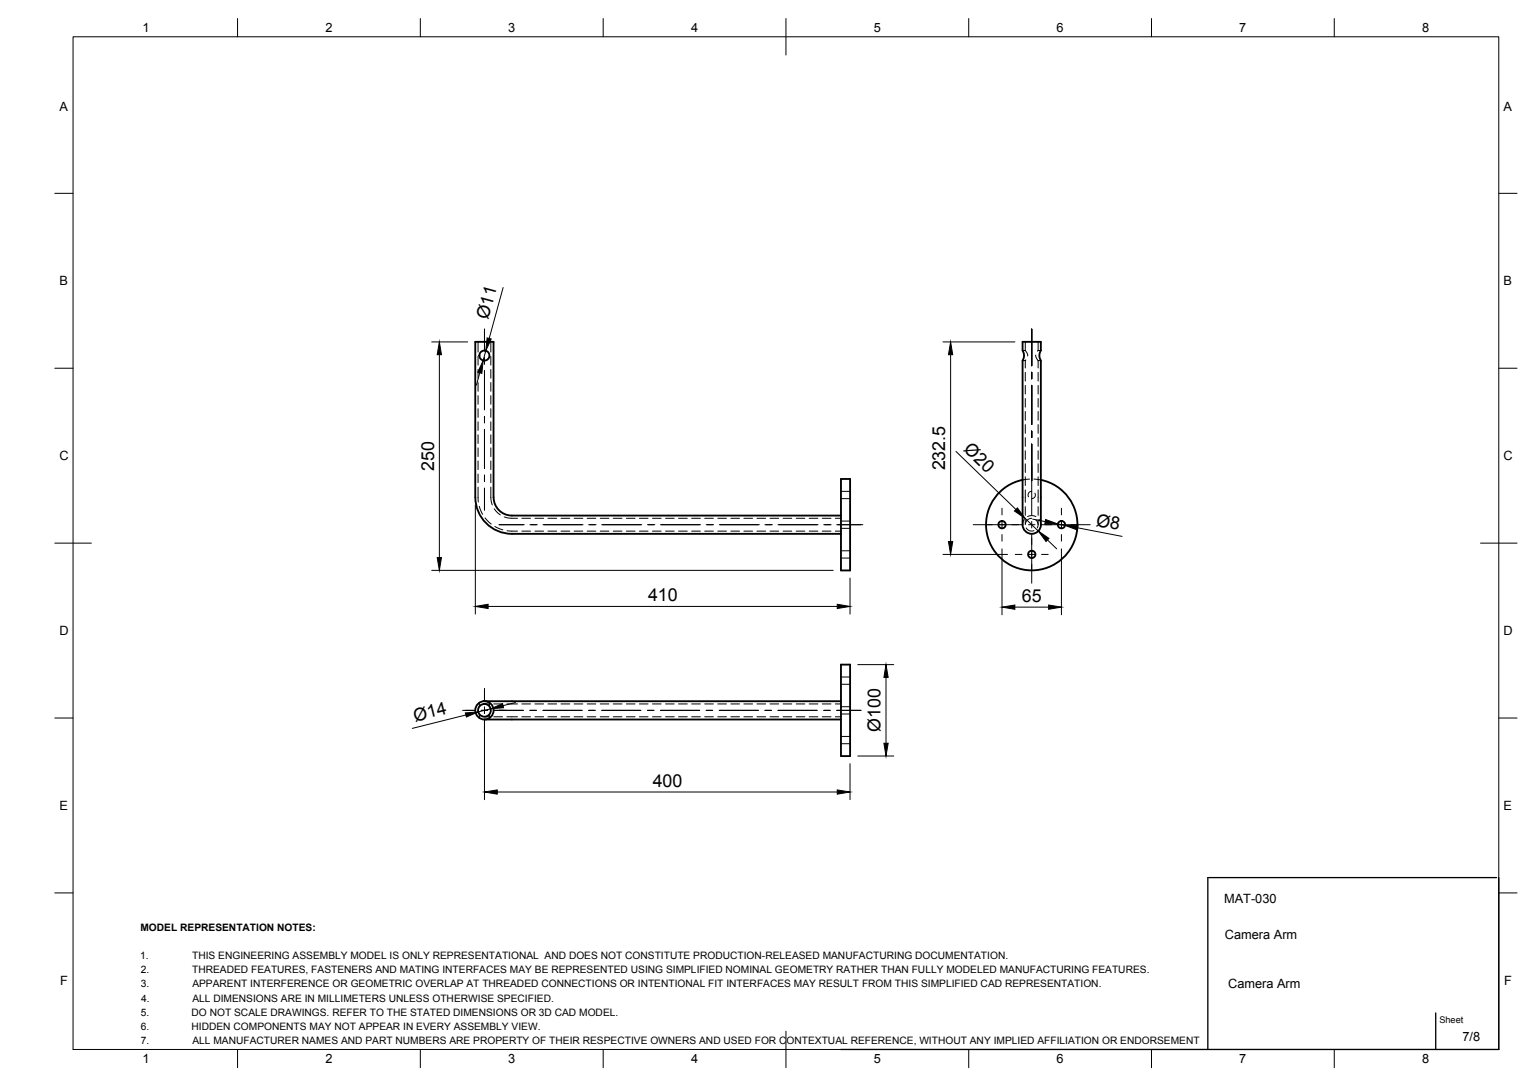
ISO-10303-21;
HEADER;
/* Generated by software containing ST-Developer
 * from STEP Tools, Inc. (www.steptools.com) 
 */

FILE_DESCRIPTION(
/* description */ ('STEP AP214'),
/* implementation_level */ '2;1');

FILE_NAME(
/* name */ 'Camera Arm.step',
/* time_stamp */ '2026-11-14T06:43:04-08:00',
/* author */ (''),
/* organization */ (''),
/* preprocessor_version */ 'ST-DEVELOPER v20.2',
/* originating_system */ 'Autodesk Translation Framework v15.17.0.0',
/* authorisation */ '');

FILE_SCHEMA (('AUTOMOTIVE_DESIGN { 1 0 10303 214 3 1 1 }'));
ENDSEC;

DATA;
#10=MECHANICAL_DESIGN_GEOMETRIC_PRESENTATION_REPRESENTATION('',(#200),#5658);
#166=B_SPLINE_CURVE_WITH_KNOTS('',3,(#4617,#4618,#4619,#4620,#4621,#4622,
#4623,#4624,#4625,#4626,#4627,#4628,#4629,#4630,#4631,#4632,#4633,#4634,
#4635,#4636,#4637,#4638,#4639,#4640,#4641,#4642,#4643,#4644,#4645,#4646,
#4647,#4648,#4649,#4650),.UNSPECIFIED.,.T.,.F.,(4,2,2,2,2,2,2,2,2,2,2,2,
2,2,2,2,4),(0.,0.212929378403861,0.425858756807722,0.637884496210834,0.849910235613946,
1.06193597501706,1.27396171442017,1.48689109282403,1.69982047122789,1.91274984963175,
2.12567922803561,2.33770496743873,2.54973070684184,2.76175644624495,2.97378218564806,
3.18671156405192,3.39964094245578),.UNSPECIFIED.);
#167=B_SPLINE_CURVE_WITH_KNOTS('',3,(#4654,#4655,#4656,#4657,#4658,#4659,
#4660,#4661,#4662,#4663,#4664,#4665,#4666,#4667,#4668,#4669,#4670,#4671,
#4672,#4673,#4674,#4675),.UNSPECIFIED.,.F.,.F.,(4,2,2,2,2,2,2,2,2,2,4),
(-1.76955541861604,-1.65739985744517,-1.5452442962743,-1.32093317393256,
-1.10285544162029,-0.884777709308018,-0.666699976995746,-0.448622244683475,
-0.224311122341738,-0.112155561170869,0.),.UNSPECIFIED.);
#168=B_SPLINE_CURVE_WITH_KNOTS('',3,(#4676,#4677,#4678,#4679,#4680,#4681,
#4682,#4683,#4684,#4685,#4686,#4687,#4688,#4689,#4690,#4691,#4692,#4693,
#4694,#4695,#4696,#4697),.UNSPECIFIED.,.F.,.F.,(4,2,2,2,2,2,2,2,2,2,4),
(-3.53911083723207,-3.4269552760612,-3.31479971489033,-3.0904885925486,
-2.87241086023632,-2.65433312792405,-2.43625539561178,-2.21817766329951,
-1.99386654095777,-1.8817109797869,-1.76955541861604),.UNSPECIFIED.);
#169=B_SPLINE_CURVE_WITH_KNOTS('',3,(#4701,#4702,#4703,#4704,#4705,#4706,
#4707,#4708,#4709,#4710,#4711,#4712,#4713,#4714,#4715,#4716,#4717,#4718,
#4719,#4720,#4721,#4722),.UNSPECIFIED.,.F.,.F.,(4,2,2,2,2,2,2,2,2,2,4),
(0.,0.112155561170869,0.224311122341738,0.448622244683475,0.666699976995746,
0.884777709308018,1.10285544162029,1.32093317393256,1.5452442962743,1.65739985744517,
1.76955541861604),.UNSPECIFIED.);
#170=B_SPLINE_CURVE_WITH_KNOTS('',3,(#4725,#4726,#4727,#4728,#4729,#4730,
#4731,#4732,#4733,#4734,#4735,#4736,#4737,#4738,#4739,#4740,#4741,#4742,
#4743,#4744,#4745,#4746,#4747,#4748,#4749,#4750,#4751,#4752,#4753,#4754,
#4755,#4756,#4757,#4758),.UNSPECIFIED.,.T.,.F.,(4,2,2,2,2,2,2,2,2,2,2,2,
2,2,2,2,4),(-3.39964094245578,-3.18671156405192,-2.97378218564806,-2.76175644624495,
-2.54973070684184,-2.33770496743873,-2.12567922803561,-1.91274984963175,
-1.69982047122789,-1.48689109282403,-1.27396171442017,-1.06193597501706,
-0.849910235613946,-0.637884496210834,-0.425858756807722,-0.212929378403861,
0.),.UNSPECIFIED.);
#171=B_SPLINE_CURVE_WITH_KNOTS('',3,(#4759,#4760,#4761,#4762,#4763,#4764,
#4765,#4766,#4767,#4768,#4769,#4770,#4771,#4772,#4773,#4774,#4775,#4776,
#4777,#4778,#4779,#4780),.UNSPECIFIED.,.F.,.F.,(4,2,2,2,2,2,2,2,2,2,4),
(1.76955541861604,1.8817109797869,1.99386654095777,2.21817766329951,2.43625539561178,
2.65433312792405,2.87241086023632,3.0904885925486,3.31479971489033,3.4269552760612,
3.53911083723207),.UNSPECIFIED.);
#172=TOROIDAL_SURFACE('',#3241,30.,7.);
#173=TOROIDAL_SURFACE('',#3245,30.,10.);
#178=SHAPE_REPRESENTATION_RELATIONSHIP('SRR','None',#5708,#189);
#189=ADVANCED_BREP_SHAPE_REPRESENTATION('',(#211),#5649);
#200=STYLED_ITEM('',(#5772),#211);
#211=MANIFOLD_SOLID_BREP('Body1',#3062);
#231=CYLINDRICAL_SURFACE('',#3249,5.50000000000001);
#232=CYLINDRICAL_SURFACE('',#3250,5.50000000000001);
#233=CYLINDRICAL_SURFACE('',#3251,4.);
#234=CYLINDRICAL_SURFACE('',#3254,4.);
#235=CYLINDRICAL_SURFACE('',#3257,4.);
#236=CYLINDRICAL_SURFACE('',#3260,4.00000000000001);
#237=CYLINDRICAL_SURFACE('',#3263,50.);
#238=CYLINDRICAL_SURFACE('',#3266,7.);
#239=CYLINDRICAL_SURFACE('',#3268,7.00000000000001);
#240=CYLINDRICAL_SURFACE('',#3270,10.);
#241=CYLINDRICAL_SURFACE('',#3272,10.);
#285=FACE_BOUND('',#566,.T.);
#286=FACE_BOUND('',#567,.T.);
#287=FACE_BOUND('',#570,.T.);
#288=FACE_BOUND('',#571,.T.);
#289=FACE_BOUND('',#573,.T.);
#290=FACE_BOUND('',#576,.T.);
#291=FACE_BOUND('',#577,.T.);
#292=FACE_BOUND('',#578,.T.);
#293=FACE_BOUND('',#579,.T.);
#294=FACE_BOUND('',#580,.T.);
#295=FACE_BOUND('',#582,.T.);
#296=FACE_BOUND('',#583,.T.);
#297=FACE_BOUND('',#584,.T.);
#298=FACE_BOUND('',#585,.T.);
#359=FACE_OUTER_BOUND('',#555,.T.);
#360=FACE_OUTER_BOUND('',#556,.T.);
#361=FACE_OUTER_BOUND('',#557,.T.);
#362=FACE_OUTER_BOUND('',#558,.T.);
#363=FACE_OUTER_BOUND('',#559,.T.);
#364=FACE_OUTER_BOUND('',#560,.T.);
#365=FACE_OUTER_BOUND('',#561,.T.);
#366=FACE_OUTER_BOUND('',#562,.T.);
#367=FACE_OUTER_BOUND('',#563,.T.);
#368=FACE_OUTER_BOUND('',#564,.T.);
#369=FACE_OUTER_BOUND('',#565,.T.);
#370=FACE_OUTER_BOUND('',#568,.T.);
#371=FACE_OUTER_BOUND('',#569,.T.);
#372=FACE_OUTER_BOUND('',#572,.T.);
#373=FACE_OUTER_BOUND('',#574,.T.);
#374=FACE_OUTER_BOUND('',#575,.T.);
#375=FACE_OUTER_BOUND('',#581,.T.);
#555=EDGE_LOOP('',(#2084,#2085,#2086,#2087));
#556=EDGE_LOOP('',(#2088,#2089,#2090,#2091));
#557=EDGE_LOOP('',(#2092,#2093,#2094,#2095,#2096));
#558=EDGE_LOOP('',(#2097,#2098,#2099,#2100,#2101));
#559=EDGE_LOOP('',(#2102,#2103,#2104,#2105));
#560=EDGE_LOOP('',(#2106,#2107,#2108,#2109));
#561=EDGE_LOOP('',(#2110,#2111,#2112,#2113));
#562=EDGE_LOOP('',(#2114,#2115,#2116,#2117));
#563=EDGE_LOOP('',(#2118,#2119,#2120,#2121));
#564=EDGE_LOOP('',(#2122,#2123,#2124,#2125));
#565=EDGE_LOOP('',(#2126,#2127,#2128,#2129));
#566=EDGE_LOOP('',(#2130,#2131));
#567=EDGE_LOOP('',(#2132,#2133));
#568=EDGE_LOOP('',(#2134,#2135,#2136,#2137));
#569=EDGE_LOOP('',(#2138,#2139,#2140,#2141));
#570=EDGE_LOOP('',(#2142));
#571=EDGE_LOOP('',(#2143));
#572=EDGE_LOOP('',(#2144));
#573=EDGE_LOOP('',(#2145));
#574=EDGE_LOOP('',(#2146));
#575=EDGE_LOOP('',(#2147));
#576=EDGE_LOOP('',(#2148));
#577=EDGE_LOOP('',(#2149));
#578=EDGE_LOOP('',(#2150));
#579=EDGE_LOOP('',(#2151));
#580=EDGE_LOOP('',(#2152));
#581=EDGE_LOOP('',(#2153));
#582=EDGE_LOOP('',(#2154));
#583=EDGE_LOOP('',(#2155));
#584=EDGE_LOOP('',(#2156));
#585=EDGE_LOOP('',(#2157));
#799=LINE('',#4652,#995);
#800=LINE('',#4724,#996);
#801=LINE('',#4785,#997);
#802=LINE('',#4791,#998);
#803=LINE('',#4797,#999);
#804=LINE('',#4803,#1000);
#805=LINE('',#4809,#1001);
#806=LINE('',#4813,#1002);
#807=LINE('',#4818,#1003);
#808=LINE('',#4822,#1004);
#809=LINE('',#4825,#1005);
#995=VECTOR('',#3705,5.50000000000001);
#996=VECTOR('',#3708,5.50000000000001);
#997=VECTOR('',#3713,4.);
#998=VECTOR('',#3720,4.);
#999=VECTOR('',#3727,4.);
#1000=VECTOR('',#3734,4.00000000000001);
#1001=VECTOR('',#3741,50.);
#1002=VECTOR('',#3746,7.);
#1003=VECTOR('',#3753,7.00000000000001);
#1004=VECTOR('',#3758,10.);
#1005=VECTOR('',#3761,10.);
#1181=CIRCLE('',#3242,7.00000000000001);
#1182=CIRCLE('',#3243,23.);
#1183=CIRCLE('',#3244,7.);
#1184=CIRCLE('',#3246,10.);
#1185=CIRCLE('',#3247,20.);
#1186=CIRCLE('',#3248,10.);
#1187=CIRCLE('',#3252,4.);
#1188=CIRCLE('',#3253,4.);
#1189=CIRCLE('',#3255,4.);
#1190=CIRCLE('',#3256,4.);
#1191=CIRCLE('',#3258,4.);
#1192=CIRCLE('',#3259,4.);
#1193=CIRCLE('',#3261,4.00000000000001);
#1194=CIRCLE('',#3262,4.00000000000001);
#1195=CIRCLE('',#3264,50.);
#1196=CIRCLE('',#3265,50.);
#1197=CIRCLE('',#3267,7.);
#1198=CIRCLE('',#3269,7.00000000000001);
#1199=CIRCLE('',#3271,10.);
#1200=CIRCLE('',#3273,10.);
#1350=VERTEX_POINT('',#4604);
#1351=VERTEX_POINT('',#4606);
#1352=VERTEX_POINT('',#4610);
#1353=VERTEX_POINT('',#4612);
#1354=VERTEX_POINT('',#4616);
#1355=VERTEX_POINT('',#4651);
#1356=VERTEX_POINT('',#4653);
#1357=VERTEX_POINT('',#4699);
#1358=VERTEX_POINT('',#4700);
#1359=VERTEX_POINT('',#4723);
#1360=VERTEX_POINT('',#4782);
#1361=VERTEX_POINT('',#4784);
#1362=VERTEX_POINT('',#4788);
#1363=VERTEX_POINT('',#4790);
#1364=VERTEX_POINT('',#4794);
#1365=VERTEX_POINT('',#4796);
#1366=VERTEX_POINT('',#4800);
#1367=VERTEX_POINT('',#4802);
#1368=VERTEX_POINT('',#4806);
#1369=VERTEX_POINT('',#4808);
#1370=VERTEX_POINT('',#4812);
#1371=VERTEX_POINT('',#4816);
#1372=VERTEX_POINT('',#4820);
#1373=VERTEX_POINT('',#4824);
#1625=EDGE_CURVE('',#1350,#1350,#1181,.T.);
#1626=EDGE_CURVE('',#1350,#1351,#1182,.T.);
#1627=EDGE_CURVE('',#1351,#1351,#1183,.T.);
#1628=EDGE_CURVE('',#1352,#1352,#1184,.T.);
#1629=EDGE_CURVE('',#1352,#1353,#1185,.T.);
#1630=EDGE_CURVE('',#1353,#1353,#1186,.T.);
#1631=EDGE_CURVE('',#1354,#1354,#166,.T.);
#1632=EDGE_CURVE('',#1354,#1355,#799,.T.);
#1633=EDGE_CURVE('',#1355,#1356,#167,.T.);
#1634=EDGE_CURVE('',#1356,#1355,#168,.T.);
#1635=EDGE_CURVE('',#1357,#1358,#169,.T.);
#1636=EDGE_CURVE('',#1358,#1359,#800,.T.);
#1637=EDGE_CURVE('',#1359,#1359,#170,.T.);
#1638=EDGE_CURVE('',#1358,#1357,#171,.T.);
#1639=EDGE_CURVE('',#1360,#1360,#1187,.T.);
#1640=EDGE_CURVE('',#1360,#1361,#801,.T.);
#1641=EDGE_CURVE('',#1361,#1361,#1188,.T.);
#1642=EDGE_CURVE('',#1362,#1362,#1189,.T.);
#1643=EDGE_CURVE('',#1362,#1363,#802,.T.);
#1644=EDGE_CURVE('',#1363,#1363,#1190,.T.);
#1645=EDGE_CURVE('',#1364,#1364,#1191,.T.);
#1646=EDGE_CURVE('',#1364,#1365,#803,.T.);
#1647=EDGE_CURVE('',#1365,#1365,#1192,.T.);
#1648=EDGE_CURVE('',#1366,#1366,#1193,.T.);
#1649=EDGE_CURVE('',#1366,#1367,#804,.T.);
#1650=EDGE_CURVE('',#1367,#1367,#1194,.T.);
#1651=EDGE_CURVE('',#1368,#1368,#1195,.T.);
#1652=EDGE_CURVE('',#1368,#1369,#805,.T.);
#1653=EDGE_CURVE('',#1369,#1369,#1196,.T.);
#1654=EDGE_CURVE('',#1351,#1370,#806,.T.);
#1655=EDGE_CURVE('',#1370,#1370,#1197,.T.);
#1656=EDGE_CURVE('',#1371,#1371,#1198,.T.);
#1657=EDGE_CURVE('',#1371,#1350,#807,.T.);
#1658=EDGE_CURVE('',#1372,#1372,#1199,.T.);
#1659=EDGE_CURVE('',#1372,#1352,#808,.T.);
#1660=EDGE_CURVE('',#1353,#1373,#809,.T.);
#1661=EDGE_CURVE('',#1373,#1373,#1200,.T.);
#2084=ORIENTED_EDGE('',*,*,#1625,.T.);
#2085=ORIENTED_EDGE('',*,*,#1626,.T.);
#2086=ORIENTED_EDGE('',*,*,#1627,.F.);
#2087=ORIENTED_EDGE('',*,*,#1626,.F.);
#2088=ORIENTED_EDGE('',*,*,#1628,.T.);
#2089=ORIENTED_EDGE('',*,*,#1629,.T.);
#2090=ORIENTED_EDGE('',*,*,#1630,.F.);
#2091=ORIENTED_EDGE('',*,*,#1629,.F.);
#2092=ORIENTED_EDGE('',*,*,#1631,.F.);
#2093=ORIENTED_EDGE('',*,*,#1632,.T.);
#2094=ORIENTED_EDGE('',*,*,#1633,.T.);
#2095=ORIENTED_EDGE('',*,*,#1634,.T.);
#2096=ORIENTED_EDGE('',*,*,#1632,.F.);
#2097=ORIENTED_EDGE('',*,*,#1635,.T.);
#2098=ORIENTED_EDGE('',*,*,#1636,.T.);
#2099=ORIENTED_EDGE('',*,*,#1637,.F.);
#2100=ORIENTED_EDGE('',*,*,#1636,.F.);
#2101=ORIENTED_EDGE('',*,*,#1638,.T.);
#2102=ORIENTED_EDGE('',*,*,#1639,.T.);
#2103=ORIENTED_EDGE('',*,*,#1640,.T.);
#2104=ORIENTED_EDGE('',*,*,#1641,.F.);
#2105=ORIENTED_EDGE('',*,*,#1640,.F.);
#2106=ORIENTED_EDGE('',*,*,#1642,.T.);
#2107=ORIENTED_EDGE('',*,*,#1643,.T.);
#2108=ORIENTED_EDGE('',*,*,#1644,.F.);
#2109=ORIENTED_EDGE('',*,*,#1643,.F.);
#2110=ORIENTED_EDGE('',*,*,#1645,.T.);
#2111=ORIENTED_EDGE('',*,*,#1646,.T.);
#2112=ORIENTED_EDGE('',*,*,#1647,.F.);
#2113=ORIENTED_EDGE('',*,*,#1646,.F.);
#2114=ORIENTED_EDGE('',*,*,#1648,.T.);
#2115=ORIENTED_EDGE('',*,*,#1649,.T.);
#2116=ORIENTED_EDGE('',*,*,#1650,.F.);
#2117=ORIENTED_EDGE('',*,*,#1649,.F.);
#2118=ORIENTED_EDGE('',*,*,#1651,.T.);
#2119=ORIENTED_EDGE('',*,*,#1652,.T.);
#2120=ORIENTED_EDGE('',*,*,#1653,.F.);
#2121=ORIENTED_EDGE('',*,*,#1652,.F.);
#2122=ORIENTED_EDGE('',*,*,#1627,.T.);
#2123=ORIENTED_EDGE('',*,*,#1654,.T.);
#2124=ORIENTED_EDGE('',*,*,#1655,.F.);
#2125=ORIENTED_EDGE('',*,*,#1654,.F.);
#2126=ORIENTED_EDGE('',*,*,#1656,.T.);
#2127=ORIENTED_EDGE('',*,*,#1657,.T.);
#2128=ORIENTED_EDGE('',*,*,#1625,.F.);
#2129=ORIENTED_EDGE('',*,*,#1657,.F.);
#2130=ORIENTED_EDGE('',*,*,#1635,.F.);
#2131=ORIENTED_EDGE('',*,*,#1638,.F.);
#2132=ORIENTED_EDGE('',*,*,#1634,.F.);
#2133=ORIENTED_EDGE('',*,*,#1633,.F.);
#2134=ORIENTED_EDGE('',*,*,#1658,.T.);
#2135=ORIENTED_EDGE('',*,*,#1659,.T.);
#2136=ORIENTED_EDGE('',*,*,#1628,.F.);
#2137=ORIENTED_EDGE('',*,*,#1659,.F.);
#2138=ORIENTED_EDGE('',*,*,#1630,.T.);
#2139=ORIENTED_EDGE('',*,*,#1660,.T.);
#2140=ORIENTED_EDGE('',*,*,#1661,.F.);
#2141=ORIENTED_EDGE('',*,*,#1660,.F.);
#2142=ORIENTED_EDGE('',*,*,#1631,.T.);
#2143=ORIENTED_EDGE('',*,*,#1637,.T.);
#2144=ORIENTED_EDGE('',*,*,#1661,.T.);
#2145=ORIENTED_EDGE('',*,*,#1656,.F.);
#2146=ORIENTED_EDGE('',*,*,#1655,.T.);
#2147=ORIENTED_EDGE('',*,*,#1653,.T.);
#2148=ORIENTED_EDGE('',*,*,#1645,.F.);
#2149=ORIENTED_EDGE('',*,*,#1639,.F.);
#2150=ORIENTED_EDGE('',*,*,#1658,.F.);
#2151=ORIENTED_EDGE('',*,*,#1642,.F.);
#2152=ORIENTED_EDGE('',*,*,#1648,.F.);
#2153=ORIENTED_EDGE('',*,*,#1651,.F.);
#2154=ORIENTED_EDGE('',*,*,#1650,.T.);
#2155=ORIENTED_EDGE('',*,*,#1647,.T.);
#2156=ORIENTED_EDGE('',*,*,#1644,.T.);
#2157=ORIENTED_EDGE('',*,*,#1641,.T.);
#2797=PLANE('',#3274);
#2798=PLANE('',#3275);
#2799=PLANE('',#3276);
#2800=PLANE('',#3277);
#2900=ADVANCED_FACE('',(#359),#172,.F.);
#2901=ADVANCED_FACE('',(#360),#173,.T.);
#2902=ADVANCED_FACE('',(#361),#231,.F.);
#2903=ADVANCED_FACE('',(#362),#232,.F.);
#2904=ADVANCED_FACE('',(#363),#233,.F.);
#2905=ADVANCED_FACE('',(#364),#234,.F.);
#2906=ADVANCED_FACE('',(#365),#235,.F.);
#2907=ADVANCED_FACE('',(#366),#236,.F.);
#2908=ADVANCED_FACE('',(#367),#237,.T.);
#2909=ADVANCED_FACE('',(#368),#238,.F.);
#2910=ADVANCED_FACE('',(#369,#285,#286),#239,.F.);
#2911=ADVANCED_FACE('',(#370),#240,.T.);
#2912=ADVANCED_FACE('',(#371,#287,#288),#241,.T.);
#2913=ADVANCED_FACE('',(#372,#289),#2797,.T.);
#2914=ADVANCED_FACE('',(#373),#2798,.T.);
#2915=ADVANCED_FACE('',(#374,#290,#291,#292,#293,#294),#2799,.T.);
#2916=ADVANCED_FACE('',(#375,#295,#296,#297,#298),#2800,.F.);
#3062=CLOSED_SHELL('',(#2900,#2901,#2902,#2903,#2904,#2905,#2906,#2907,
#2908,#2909,#2910,#2911,#2912,#2913,#2914,#2915,#2916));
#3240=AXIS2_PLACEMENT_3D('',#4602,#3685,#3686);
#3241=AXIS2_PLACEMENT_3D('',#4603,#3687,#3688);
#3242=AXIS2_PLACEMENT_3D('',#4605,#3689,#3690);
#3243=AXIS2_PLACEMENT_3D('',#4607,#3691,#3692);
#3244=AXIS2_PLACEMENT_3D('',#4608,#3693,#3694);
#3245=AXIS2_PLACEMENT_3D('',#4609,#3695,#3696);
#3246=AXIS2_PLACEMENT_3D('',#4611,#3697,#3698);
#3247=AXIS2_PLACEMENT_3D('',#4613,#3699,#3700);
#3248=AXIS2_PLACEMENT_3D('',#4614,#3701,#3702);
#3249=AXIS2_PLACEMENT_3D('',#4615,#3703,#3704);
#3250=AXIS2_PLACEMENT_3D('',#4698,#3706,#3707);
#3251=AXIS2_PLACEMENT_3D('',#4781,#3709,#3710);
#3252=AXIS2_PLACEMENT_3D('',#4783,#3711,#3712);
#3253=AXIS2_PLACEMENT_3D('',#4786,#3714,#3715);
#3254=AXIS2_PLACEMENT_3D('',#4787,#3716,#3717);
#3255=AXIS2_PLACEMENT_3D('',#4789,#3718,#3719);
#3256=AXIS2_PLACEMENT_3D('',#4792,#3721,#3722);
#3257=AXIS2_PLACEMENT_3D('',#4793,#3723,#3724);
#3258=AXIS2_PLACEMENT_3D('',#4795,#3725,#3726);
#3259=AXIS2_PLACEMENT_3D('',#4798,#3728,#3729);
#3260=AXIS2_PLACEMENT_3D('',#4799,#3730,#3731);
#3261=AXIS2_PLACEMENT_3D('',#4801,#3732,#3733);
#3262=AXIS2_PLACEMENT_3D('',#4804,#3735,#3736);
#3263=AXIS2_PLACEMENT_3D('',#4805,#3737,#3738);
#3264=AXIS2_PLACEMENT_3D('',#4807,#3739,#3740);
#3265=AXIS2_PLACEMENT_3D('',#4810,#3742,#3743);
#3266=AXIS2_PLACEMENT_3D('',#4811,#3744,#3745);
#3267=AXIS2_PLACEMENT_3D('',#4814,#3747,#3748);
#3268=AXIS2_PLACEMENT_3D('',#4815,#3749,#3750);
#3269=AXIS2_PLACEMENT_3D('',#4817,#3751,#3752);
#3270=AXIS2_PLACEMENT_3D('',#4819,#3754,#3755);
#3271=AXIS2_PLACEMENT_3D('',#4821,#3756,#3757);
#3272=AXIS2_PLACEMENT_3D('',#4823,#3759,#3760);
#3273=AXIS2_PLACEMENT_3D('',#4826,#3762,#3763);
#3274=AXIS2_PLACEMENT_3D('',#4827,#3764,#3765);
#3275=AXIS2_PLACEMENT_3D('',#4828,#3766,#3767);
#3276=AXIS2_PLACEMENT_3D('',#4829,#3768,#3769);
#3277=AXIS2_PLACEMENT_3D('',#4830,#3770,#3771);
#3685=DIRECTION('axis',(0.,0.,1.));
#3686=DIRECTION('refdir',(1.,0.,0.));
#3687=DIRECTION('center_axis',(-1.,0.,0.));
#3688=DIRECTION('ref_axis',(0.,0.,1.));
#3689=DIRECTION('center_axis',(0.,-1.,0.));
#3690=DIRECTION('ref_axis',(0.,0.,1.));
#3691=DIRECTION('center_axis',(-1.,0.,0.));
#3692=DIRECTION('ref_axis',(0.,0.,1.));
#3693=DIRECTION('center_axis',(0.,-6.12323399573677E-17,1.));
#3694=DIRECTION('ref_axis',(0.,-1.,-6.12323399573677E-17));
#3695=DIRECTION('center_axis',(-1.,0.,0.));
#3696=DIRECTION('ref_axis',(0.,0.,1.));
#3697=DIRECTION('center_axis',(0.,0.,1.));
#3698=DIRECTION('ref_axis',(1.,0.,0.));
#3699=DIRECTION('center_axis',(1.,0.,0.));
#3700=DIRECTION('ref_axis',(0.,0.,1.));
#3701=DIRECTION('center_axis',(0.,-1.,4.68844182696434E-17));
#3702=DIRECTION('ref_axis',(1.,0.,0.));
#3703=DIRECTION('center_axis',(1.,0.,0.));
#3704=DIRECTION('ref_axis',(0.,0.,-1.));
#3705=DIRECTION('',(1.,0.,0.));
#3706=DIRECTION('center_axis',(1.,0.,0.));
#3707=DIRECTION('ref_axis',(0.,0.,-1.));
#3708=DIRECTION('',(1.,0.,0.));
#3709=DIRECTION('center_axis',(0.,0.,-1.));
#3710=DIRECTION('ref_axis',(-1.,0.,0.));
#3711=DIRECTION('center_axis',(0.,0.,1.));
#3712=DIRECTION('ref_axis',(1.,0.,0.));
#3713=DIRECTION('',(0.,0.,-1.));
#3714=DIRECTION('center_axis',(0.,0.,1.));
#3715=DIRECTION('ref_axis',(1.,0.,0.));
#3716=DIRECTION('center_axis',(0.,0.,-1.));
#3717=DIRECTION('ref_axis',(-1.,0.,0.));
#3718=DIRECTION('center_axis',(0.,0.,1.));
#3719=DIRECTION('ref_axis',(1.,0.,0.));
#3720=DIRECTION('',(0.,0.,-1.));
#3721=DIRECTION('center_axis',(0.,0.,1.));
#3722=DIRECTION('ref_axis',(1.,0.,0.));
#3723=DIRECTION('center_axis',(0.,0.,-1.));
#3724=DIRECTION('ref_axis',(-1.,0.,0.));
#3725=DIRECTION('center_axis',(0.,0.,1.));
#3726=DIRECTION('ref_axis',(1.,0.,0.));
#3727=DIRECTION('',(0.,0.,-1.));
#3728=DIRECTION('center_axis',(0.,0.,1.));
#3729=DIRECTION('ref_axis',(1.,0.,0.));
#3730=DIRECTION('center_axis',(0.,0.,-1.));
#3731=DIRECTION('ref_axis',(-1.,0.,0.));
#3732=DIRECTION('center_axis',(0.,0.,1.));
#3733=DIRECTION('ref_axis',(1.,0.,0.));
#3734=DIRECTION('',(0.,0.,-1.));
#3735=DIRECTION('center_axis',(0.,0.,1.));
#3736=DIRECTION('ref_axis',(1.,0.,0.));
#3737=DIRECTION('center_axis',(0.,0.,-1.));
#3738=DIRECTION('ref_axis',(-1.,0.,0.));
#3739=DIRECTION('center_axis',(0.,0.,1.));
#3740=DIRECTION('ref_axis',(1.,0.,0.));
#3741=DIRECTION('',(0.,0.,1.));
#3742=DIRECTION('center_axis',(0.,0.,1.));
#3743=DIRECTION('ref_axis',(1.,0.,0.));
#3744=DIRECTION('center_axis',(0.,4.68844182696434E-17,-1.));
#3745=DIRECTION('ref_axis',(0.,1.,4.68844182696434E-17));
#3746=DIRECTION('',(0.,4.68844182696434E-17,-1.));
#3747=DIRECTION('center_axis',(0.,0.,1.));
#3748=DIRECTION('ref_axis',(1.,0.,0.));
#3749=DIRECTION('center_axis',(0.,1.,0.));
#3750=DIRECTION('ref_axis',(0.,0.,1.));
#3751=DIRECTION('center_axis',(0.,-1.,4.68844182696434E-17));
#3752=DIRECTION('ref_axis',(0.,-4.68844182696434E-17,-1.));
#3753=DIRECTION('',(0.,1.,0.));
#3754=DIRECTION('center_axis',(0.,4.68844182696434E-17,-1.));
#3755=DIRECTION('ref_axis',(0.,1.,4.68844182696434E-17));
#3756=DIRECTION('center_axis',(0.,0.,1.));
#3757=DIRECTION('ref_axis',(1.,0.,0.));
#3758=DIRECTION('',(0.,-4.68844182696434E-17,1.));
#3759=DIRECTION('center_axis',(0.,1.,0.));
#3760=DIRECTION('ref_axis',(0.,0.,1.));
#3761=DIRECTION('',(0.,-1.,0.));
#3762=DIRECTION('center_axis',(0.,-1.,4.68844182696434E-17));
#3763=DIRECTION('ref_axis',(1.,0.,0.));
#3764=DIRECTION('center_axis',(0.,-1.,4.68844182696434E-17));
#3765=DIRECTION('ref_axis',(1.,0.,0.));
#3766=DIRECTION('center_axis',(0.,0.,1.));
#3767=DIRECTION('ref_axis',(1.,0.,0.));
#3768=DIRECTION('center_axis',(0.,0.,1.));
#3769=DIRECTION('ref_axis',(1.,0.,0.));
#3770=DIRECTION('center_axis',(0.,0.,1.));
#3771=DIRECTION('ref_axis',(1.,0.,0.));
#4602=CARTESIAN_POINT('',(0.,0.,0.));
#4603=CARTESIAN_POINT('Origin',(0.,-30.,370.));
#4604=CARTESIAN_POINT('',(8.57252759403147E-16,-30.,393.));
#4605=CARTESIAN_POINT('Origin',(0.,-30.,400.));
#4606=CARTESIAN_POINT('',(8.57252759403147E-16,-6.99999999999999,370.));
#4607=CARTESIAN_POINT('Origin',(8.57252759403147E-16,-30.,370.));
#4608=CARTESIAN_POINT('Origin',(0.,1.04083408558608E-14,370.));
#4609=CARTESIAN_POINT('Origin',(0.,-30.,370.));
#4610=CARTESIAN_POINT('',(1.22464679914735E-15,-10.,370.));
#4611=CARTESIAN_POINT('Origin',(0.,-3.46944695195361E-15,370.));
#4612=CARTESIAN_POINT('',(1.22464679914735E-15,-30.,390.));
#4613=CARTESIAN_POINT('Origin',(1.22464679914735E-15,-30.,370.));
#4614=CARTESIAN_POINT('Origin',(0.,-30.,400.));
#4615=CARTESIAN_POINT('Origin',(-50.,-185.,400.));
#4616=CARTESIAN_POINT('',(-8.35164654424502,-185.,405.5));
#4617=CARTESIAN_POINT('Ctrl Pts',(-8.35164654424504,-185.,394.5));
#4618=CARTESIAN_POINT('Ctrl Pts',(-8.35164654424504,-184.290235405321,394.5));
#4619=CARTESIAN_POINT('Ctrl Pts',(-8.45174305106268,-183.547853071563,394.64504316336));
#4620=CARTESIAN_POINT('Ctrl Pts',(-8.78438651561337,-182.199599169859,395.210212504666));
#4621=CARTESIAN_POINT('Ctrl Pts',(-9.00975031605896,-181.591824169425,395.630001237523));
#4622=CARTESIAN_POINT('Ctrl Pts',(-9.41491390301225,-180.632042150617,396.589783256331));
#4623=CARTESIAN_POINT('Ctrl Pts',(-9.62434109787453,-180.210790188028,397.198189638843));
#4624=CARTESIAN_POINT('Ctrl Pts',(-9.91836499005242,-179.644390383362,398.549441755203));
#4625=CARTESIAN_POINT('Ctrl Pts',(-10.,-179.5,399.293247535323));
#4626=CARTESIAN_POINT('Ctrl Pts',(-10.,-179.5,400.706752464677));
#4627=CARTESIAN_POINT('Ctrl Pts',(-9.91836499005242,-179.644390383362,401.450558244797));
#4628=CARTESIAN_POINT('Ctrl Pts',(-9.62434109787453,-180.210790188028,402.801810361157));
#4629=CARTESIAN_POINT('Ctrl Pts',(-9.41491390301225,-180.632042150617,403.410216743669));
#4630=CARTESIAN_POINT('Ctrl Pts',(-9.00975031605896,-181.591824169425,404.369998762477));
#4631=CARTESIAN_POINT('Ctrl Pts',(-8.78438651561337,-182.199599169859,404.789787495334));
#4632=CARTESIAN_POINT('Ctrl Pts',(-8.45174305106268,-183.547853071563,405.35495683664));
#4633=CARTESIAN_POINT('Ctrl Pts',(-8.35164654424506,-184.290235405321,405.5));
#4634=CARTESIAN_POINT('Ctrl Pts',(-8.35164654424506,-185.70976459468,405.5));
#4635=CARTESIAN_POINT('Ctrl Pts',(-8.45174305106268,-186.452146928437,405.35495683664));
#4636=CARTESIAN_POINT('Ctrl Pts',(-8.78438651561337,-187.800400830141,404.789787495334));
#4637=CARTESIAN_POINT('Ctrl Pts',(-9.00975031605896,-188.408175830575,404.369998762477));
#4638=CARTESIAN_POINT('Ctrl Pts',(-9.41491390301225,-189.367957849383,403.410216743669));
#4639=CARTESIAN_POINT('Ctrl Pts',(-9.62434109787455,-189.789209811972,402.801810361157));
#4640=CARTESIAN_POINT('Ctrl Pts',(-9.91836499005243,-190.355609616638,401.450558244797));
#4641=CARTESIAN_POINT('Ctrl Pts',(-10.,-190.5,400.706752464677));
#4642=CARTESIAN_POINT('Ctrl Pts',(-10.,-190.5,399.293247535323));
#4643=CARTESIAN_POINT('Ctrl Pts',(-9.9183649900524,-190.355609616638,398.549441755203));
#4644=CARTESIAN_POINT('Ctrl Pts',(-9.62434109787451,-189.789209811972,397.198189638843));
#4645=CARTESIAN_POINT('Ctrl Pts',(-9.41491390301225,-189.367957849383,396.589783256331));
#4646=CARTESIAN_POINT('Ctrl Pts',(-9.00975031605896,-188.408175830575,395.630001237523));
#4647=CARTESIAN_POINT('Ctrl Pts',(-8.78438651561337,-187.800400830141,395.210212504666));
#4648=CARTESIAN_POINT('Ctrl Pts',(-8.45174305106268,-186.452146928437,394.64504316336));
#4649=CARTESIAN_POINT('Ctrl Pts',(-8.35164654424504,-185.70976459468,394.5));
#4650=CARTESIAN_POINT('Ctrl Pts',(-8.35164654424504,-185.,394.5));
#4651=CARTESIAN_POINT('',(-4.33012701892219,-185.,405.5));
#4652=CARTESIAN_POINT('',(-50.,-185.,405.5));
#4653=CARTESIAN_POINT('',(-4.33012701892219,-185.,394.5));
#4654=CARTESIAN_POINT('Ctrl Pts',(-4.33012701892219,-185.,405.5));
#4655=CARTESIAN_POINT('Ctrl Pts',(-4.33012701892219,-185.37385187057,405.5));
#4656=CARTESIAN_POINT('Ctrl Pts',(-4.37998128622333,-185.746075739511,405.461618176925));
#4657=CARTESIAN_POINT('Ctrl Pts',(-4.55888740591996,-186.468280486434,405.313196276448));
#4658=CARTESIAN_POINT('Ctrl Pts',(-4.68703690659531,-186.81849775152,405.203220220576));
#4659=CARTESIAN_POINT('Ctrl Pts',(-5.13065352868785,-187.815687292683,404.779503215329));
#4660=CARTESIAN_POINT('Ctrl Pts',(-5.50080088534137,-188.411054784548,404.367119808505));
#4661=CARTESIAN_POINT('Ctrl Pts',(-6.13076939848926,-189.353835745446,403.424338847606));
#4662=CARTESIAN_POINT('Ctrl Pts',(-6.44230837852261,-189.773691234096,402.828149962177));
#4663=CARTESIAN_POINT('Ctrl Pts',(-6.87828608217357,-190.347486404219,401.48018651652));
#4664=CARTESIAN_POINT('Ctrl Pts',(-7.00000000000001,-190.5,400.726925774374));
#4665=CARTESIAN_POINT('Ctrl Pts',(-7.00000000000001,-190.5,399.273074225626));
#4666=CARTESIAN_POINT('Ctrl Pts',(-6.87828608217358,-190.347486404219,398.51981348348));
#4667=CARTESIAN_POINT('Ctrl Pts',(-6.44230837852261,-189.773691234096,397.171850037823));
#4668=CARTESIAN_POINT('Ctrl Pts',(-6.13076939848926,-189.353835745446,396.575661152394));
#4669=CARTESIAN_POINT('Ctrl Pts',(-5.50080088534137,-188.411054784548,395.632880191495));
#4670=CARTESIAN_POINT('Ctrl Pts',(-5.13065352868785,-187.815687292683,395.220496784671));
#4671=CARTESIAN_POINT('Ctrl Pts',(-4.68703690659531,-186.81849775152,394.796779779424));
#4672=CARTESIAN_POINT('Ctrl Pts',(-4.55888740591996,-186.468280486434,394.686803723552));
#4673=CARTESIAN_POINT('Ctrl Pts',(-4.37998128622333,-185.746075739511,394.538381823075));
#4674=CARTESIAN_POINT('Ctrl Pts',(-4.3301270189222,-185.37385187057,394.5));
#4675=CARTESIAN_POINT('Ctrl Pts',(-4.3301270189222,-185.,394.5));
#4676=CARTESIAN_POINT('Ctrl Pts',(-4.3301270189222,-185.,394.5));
#4677=CARTESIAN_POINT('Ctrl Pts',(-4.3301270189222,-184.626148129431,394.5));
#4678=CARTESIAN_POINT('Ctrl Pts',(-4.37998128622333,-184.25392426049,394.538381823075));
#4679=CARTESIAN_POINT('Ctrl Pts',(-4.55888740591996,-183.531719513566,394.686803723552));
#4680=CARTESIAN_POINT('Ctrl Pts',(-4.68703690659531,-183.18150224848,394.796779779424));
#4681=CARTESIAN_POINT('Ctrl Pts',(-5.13065352868785,-182.184312707317,395.220496784671));
#4682=CARTESIAN_POINT('Ctrl Pts',(-5.50080088534137,-181.588945215453,395.632880191495));
#4683=CARTESIAN_POINT('Ctrl Pts',(-6.13076939848926,-180.646164254554,396.575661152394));
#4684=CARTESIAN_POINT('Ctrl Pts',(-6.44230837852252,-180.226308765904,397.171850037822));
#4685=CARTESIAN_POINT('Ctrl Pts',(-6.87828608217351,-179.652513595781,398.51981348348));
#4686=CARTESIAN_POINT('Ctrl Pts',(-7.00000000000001,-179.5,399.273074225626));
#4687=CARTESIAN_POINT('Ctrl Pts',(-7.00000000000001,-179.5,400.726925774374));
#4688=CARTESIAN_POINT('Ctrl Pts',(-6.87828608217354,-179.652513595781,401.48018651652));
#4689=CARTESIAN_POINT('Ctrl Pts',(-6.44230837852263,-180.226308765904,402.828149962177));
#4690=CARTESIAN_POINT('Ctrl Pts',(-6.13076939848926,-180.646164254554,403.424338847606));
#4691=CARTESIAN_POINT('Ctrl Pts',(-5.50080088534137,-181.588945215453,404.367119808505));
#4692=CARTESIAN_POINT('Ctrl Pts',(-5.13065352868785,-182.184312707317,404.779503215329));
#4693=CARTESIAN_POINT('Ctrl Pts',(-4.68703690659531,-183.18150224848,405.203220220576));
#4694=CARTESIAN_POINT('Ctrl Pts',(-4.55888740591996,-183.531719513566,405.313196276448));
#4695=CARTESIAN_POINT('Ctrl Pts',(-4.37998128622333,-184.25392426049,405.461618176925));
#4696=CARTESIAN_POINT('Ctrl Pts',(-4.33012701892219,-184.626148129431,405.5));
#4697=CARTESIAN_POINT('Ctrl Pts',(-4.33012701892219,-185.,405.5));
#4698=CARTESIAN_POINT('Origin',(-50.,-185.,400.));
#4699=CARTESIAN_POINT('',(4.33012701892219,-185.,394.5));
#4700=CARTESIAN_POINT('',(4.3301270189222,-185.,405.5));
#4701=CARTESIAN_POINT('Ctrl Pts',(4.3301270189222,-185.,394.5));
#4702=CARTESIAN_POINT('Ctrl Pts',(4.3301270189222,-185.37385187057,394.5));
#4703=CARTESIAN_POINT('Ctrl Pts',(4.37998128622333,-185.746075739511,394.538381823075));
#4704=CARTESIAN_POINT('Ctrl Pts',(4.55888740591996,-186.468280486434,394.686803723552));
#4705=CARTESIAN_POINT('Ctrl Pts',(4.68703690659531,-186.81849775152,394.796779779424));
#4706=CARTESIAN_POINT('Ctrl Pts',(5.13065352868785,-187.815687292683,395.220496784671));
#4707=CARTESIAN_POINT('Ctrl Pts',(5.50080088534137,-188.411054784548,395.632880191495));
#4708=CARTESIAN_POINT('Ctrl Pts',(6.13076939848926,-189.353835745446,396.575661152394));
#4709=CARTESIAN_POINT('Ctrl Pts',(6.44230837852261,-189.773691234096,397.171850037823));
#4710=CARTESIAN_POINT('Ctrl Pts',(6.87828608217358,-190.347486404219,398.51981348348));
#4711=CARTESIAN_POINT('Ctrl Pts',(7.00000000000001,-190.5,399.273074225626));
#4712=CARTESIAN_POINT('Ctrl Pts',(7.00000000000001,-190.5,400.726925774374));
#4713=CARTESIAN_POINT('Ctrl Pts',(6.87828608217357,-190.347486404219,401.48018651652));
#4714=CARTESIAN_POINT('Ctrl Pts',(6.44230837852261,-189.773691234096,402.828149962177));
#4715=CARTESIAN_POINT('Ctrl Pts',(6.13076939848926,-189.353835745446,403.424338847606));
#4716=CARTESIAN_POINT('Ctrl Pts',(5.50080088534137,-188.411054784548,404.367119808505));
#4717=CARTESIAN_POINT('Ctrl Pts',(5.13065352868785,-187.815687292683,404.779503215329));
#4718=CARTESIAN_POINT('Ctrl Pts',(4.68703690659531,-186.81849775152,405.203220220576));
#4719=CARTESIAN_POINT('Ctrl Pts',(4.55888740591996,-186.468280486434,405.313196276448));
#4720=CARTESIAN_POINT('Ctrl Pts',(4.37998128622333,-185.746075739511,405.461618176925));
#4721=CARTESIAN_POINT('Ctrl Pts',(4.33012701892219,-185.37385187057,405.5));
#4722=CARTESIAN_POINT('Ctrl Pts',(4.33012701892219,-185.,405.5));
#4723=CARTESIAN_POINT('',(8.35164654424502,-185.,405.5));
#4724=CARTESIAN_POINT('',(-50.,-185.,405.5));
#4725=CARTESIAN_POINT('Ctrl Pts',(8.35164654424504,-185.,394.5));
#4726=CARTESIAN_POINT('Ctrl Pts',(8.35164654424504,-185.70976459468,394.5));
#4727=CARTESIAN_POINT('Ctrl Pts',(8.45174305106268,-186.452146928437,394.64504316336));
#4728=CARTESIAN_POINT('Ctrl Pts',(8.78438651561337,-187.800400830141,395.210212504666));
#4729=CARTESIAN_POINT('Ctrl Pts',(9.00975031605896,-188.408175830575,395.630001237523));
#4730=CARTESIAN_POINT('Ctrl Pts',(9.41491390301225,-189.367957849383,396.589783256331));
#4731=CARTESIAN_POINT('Ctrl Pts',(9.62434109787451,-189.789209811972,397.198189638843));
#4732=CARTESIAN_POINT('Ctrl Pts',(9.9183649900524,-190.355609616638,398.549441755203));
#4733=CARTESIAN_POINT('Ctrl Pts',(10.,-190.5,399.293247535323));
#4734=CARTESIAN_POINT('Ctrl Pts',(10.,-190.5,400.706752464677));
#4735=CARTESIAN_POINT('Ctrl Pts',(9.91836499005243,-190.355609616638,401.450558244797));
#4736=CARTESIAN_POINT('Ctrl Pts',(9.62434109787455,-189.789209811972,402.801810361157));
#4737=CARTESIAN_POINT('Ctrl Pts',(9.41491390301225,-189.367957849383,403.410216743669));
#4738=CARTESIAN_POINT('Ctrl Pts',(9.00975031605896,-188.408175830575,404.369998762477));
#4739=CARTESIAN_POINT('Ctrl Pts',(8.78438651561337,-187.800400830141,404.789787495334));
#4740=CARTESIAN_POINT('Ctrl Pts',(8.45174305106268,-186.452146928437,405.35495683664));
#4741=CARTESIAN_POINT('Ctrl Pts',(8.35164654424506,-185.70976459468,405.5));
#4742=CARTESIAN_POINT('Ctrl Pts',(8.35164654424506,-184.290235405321,405.5));
#4743=CARTESIAN_POINT('Ctrl Pts',(8.45174305106268,-183.547853071563,405.35495683664));
#4744=CARTESIAN_POINT('Ctrl Pts',(8.78438651561337,-182.199599169859,404.789787495334));
#4745=CARTESIAN_POINT('Ctrl Pts',(9.00975031605896,-181.591824169425,404.369998762477));
#4746=CARTESIAN_POINT('Ctrl Pts',(9.41491390301225,-180.632042150617,403.410216743669));
#4747=CARTESIAN_POINT('Ctrl Pts',(9.62434109787453,-180.210790188028,402.801810361157));
#4748=CARTESIAN_POINT('Ctrl Pts',(9.91836499005242,-179.644390383362,401.450558244797));
#4749=CARTESIAN_POINT('Ctrl Pts',(10.,-179.5,400.706752464677));
#4750=CARTESIAN_POINT('Ctrl Pts',(10.,-179.5,399.293247535323));
#4751=CARTESIAN_POINT('Ctrl Pts',(9.91836499005242,-179.644390383362,398.549441755203));
#4752=CARTESIAN_POINT('Ctrl Pts',(9.62434109787453,-180.210790188028,397.198189638843));
#4753=CARTESIAN_POINT('Ctrl Pts',(9.41491390301225,-180.632042150617,396.589783256331));
#4754=CARTESIAN_POINT('Ctrl Pts',(9.00975031605896,-181.591824169425,395.630001237523));
#4755=CARTESIAN_POINT('Ctrl Pts',(8.78438651561337,-182.199599169859,395.210212504666));
#4756=CARTESIAN_POINT('Ctrl Pts',(8.45174305106268,-183.547853071563,394.64504316336));
#4757=CARTESIAN_POINT('Ctrl Pts',(8.35164654424504,-184.290235405321,394.5));
#4758=CARTESIAN_POINT('Ctrl Pts',(8.35164654424504,-185.,394.5));
#4759=CARTESIAN_POINT('Ctrl Pts',(4.33012701892219,-185.,405.5));
#4760=CARTESIAN_POINT('Ctrl Pts',(4.33012701892219,-184.626148129431,405.5));
#4761=CARTESIAN_POINT('Ctrl Pts',(4.37998128622333,-184.25392426049,405.461618176925));
#4762=CARTESIAN_POINT('Ctrl Pts',(4.55888740591996,-183.531719513566,405.313196276448));
#4763=CARTESIAN_POINT('Ctrl Pts',(4.68703690659531,-183.18150224848,405.203220220576));
#4764=CARTESIAN_POINT('Ctrl Pts',(5.13065352868785,-182.184312707317,404.779503215329));
#4765=CARTESIAN_POINT('Ctrl Pts',(5.50080088534137,-181.588945215453,404.367119808505));
#4766=CARTESIAN_POINT('Ctrl Pts',(6.13076939848926,-180.646164254554,403.424338847606));
#4767=CARTESIAN_POINT('Ctrl Pts',(6.44230837852263,-180.226308765904,402.828149962177));
#4768=CARTESIAN_POINT('Ctrl Pts',(6.87828608217354,-179.652513595781,401.48018651652));
#4769=CARTESIAN_POINT('Ctrl Pts',(7.00000000000001,-179.5,400.726925774374));
#4770=CARTESIAN_POINT('Ctrl Pts',(7.00000000000001,-179.5,399.273074225626));
#4771=CARTESIAN_POINT('Ctrl Pts',(6.87828608217351,-179.652513595781,398.51981348348));
#4772=CARTESIAN_POINT('Ctrl Pts',(6.44230837852252,-180.226308765904,397.171850037822));
#4773=CARTESIAN_POINT('Ctrl Pts',(6.13076939848926,-180.646164254554,396.575661152394));
#4774=CARTESIAN_POINT('Ctrl Pts',(5.50080088534137,-181.588945215453,395.632880191495));
#4775=CARTESIAN_POINT('Ctrl Pts',(5.13065352868785,-182.184312707317,395.220496784671));
#4776=CARTESIAN_POINT('Ctrl Pts',(4.68703690659531,-183.18150224848,394.796779779424));
#4777=CARTESIAN_POINT('Ctrl Pts',(4.55888740591996,-183.531719513566,394.686803723552));
#4778=CARTESIAN_POINT('Ctrl Pts',(4.37998128622333,-184.25392426049,394.538381823075));
#4779=CARTESIAN_POINT('Ctrl Pts',(4.3301270189222,-184.626148129431,394.5));
#4780=CARTESIAN_POINT('Ctrl Pts',(4.3301270189222,-185.,394.5));
#4781=CARTESIAN_POINT('Origin',(-32.5,3.40419430537205E-13,10.));
#4782=CARTESIAN_POINT('',(-28.5,3.39929571817546E-13,10.));
#4783=CARTESIAN_POINT('Origin',(-32.5,3.40419430537205E-13,10.));
#4784=CARTESIAN_POINT('',(-28.5,3.39929571817546E-13,0.));
#4785=CARTESIAN_POINT('',(-28.5,3.39929571817546E-13,10.));
#4786=CARTESIAN_POINT('Origin',(-32.5,3.40419430537205E-13,0.));
#4787=CARTESIAN_POINT('Origin',(-2.26946287024804E-13,-32.5,10.));
#4788=CARTESIAN_POINT('',(3.99999999999977,-32.5,10.));
#4789=CARTESIAN_POINT('Origin',(-2.26946287024804E-13,-32.5,10.));
#4790=CARTESIAN_POINT('',(3.99999999999977,-32.5,0.));
#4791=CARTESIAN_POINT('',(3.99999999999977,-32.5,10.));
#4792=CARTESIAN_POINT('Origin',(-2.26946287024804E-13,-32.5,0.));
#4793=CARTESIAN_POINT('Origin',(32.5,-1.13473143512402E-13,10.));
#4794=CARTESIAN_POINT('',(36.5,-1.13963002232061E-13,10.));
#4795=CARTESIAN_POINT('Origin',(32.5,-1.13473143512402E-13,10.));
#4796=CARTESIAN_POINT('',(36.5,-1.13963002232061E-13,0.));
#4797=CARTESIAN_POINT('',(36.5,-1.13963002232061E-13,10.));
#4798=CARTESIAN_POINT('Origin',(32.5,-1.13473143512402E-13,0.));
#4799=CARTESIAN_POINT('Origin',(0.,32.5,10.));
#4800=CARTESIAN_POINT('',(4.00000000000001,32.5,10.));
#4801=CARTESIAN_POINT('Origin',(0.,32.5,10.));
#4802=CARTESIAN_POINT('',(4.00000000000001,32.5,0.));
#4803=CARTESIAN_POINT('',(4.00000000000001,32.5,10.));
#4804=CARTESIAN_POINT('Origin',(0.,32.5,0.));
#4805=CARTESIAN_POINT('Origin',(0.,-1.73472347597681E-14,10.));
#4806=CARTESIAN_POINT('',(50.,-2.34704687555048E-14,0.));
#4807=CARTESIAN_POINT('Origin',(0.,-1.73472347597681E-14,0.));
#4808=CARTESIAN_POINT('',(50.,-2.34704687555048E-14,10.));
#4809=CARTESIAN_POINT('',(50.,-2.34704687555048E-14,10.));
#4810=CARTESIAN_POINT('Origin',(0.,-1.73472347597681E-14,10.));
#4811=CARTESIAN_POINT('Origin',(0.,-1.73472347597681E-14,370.));
#4812=CARTESIAN_POINT('',(-8.57252759403147E-16,-7.,10.));
#4813=CARTESIAN_POINT('',(-8.57252759403147E-16,-7.00000000000002,370.));
#4814=CARTESIAN_POINT('Origin',(0.,-4.68844182696437E-16,10.));
#4815=CARTESIAN_POINT('Origin',(0.,-200.,400.));
#4816=CARTESIAN_POINT('',(-8.57252759403148E-16,-200.,393.));
#4817=CARTESIAN_POINT('Origin',(0.,-200.,400.));
#4818=CARTESIAN_POINT('',(-8.57252759403148E-16,-200.,393.));
#4819=CARTESIAN_POINT('Origin',(0.,-1.73472347597681E-14,370.));
#4820=CARTESIAN_POINT('',(-1.22464679914735E-15,-10.,10.));
#4821=CARTESIAN_POINT('Origin',(0.,-4.68844182696437E-16,10.));
#4822=CARTESIAN_POINT('',(-1.22464679914735E-15,-10.,370.));
#4823=CARTESIAN_POINT('Origin',(0.,-200.,400.));
#4824=CARTESIAN_POINT('',(-1.22464679914735E-15,-200.,390.));
#4825=CARTESIAN_POINT('',(-1.22464679914735E-15,-200.,390.));
#4826=CARTESIAN_POINT('Origin',(0.,-200.,400.));
#4827=CARTESIAN_POINT('Origin',(0.,-200.,400.));
#4828=CARTESIAN_POINT('Origin',(0.,-1.73472347597681E-14,10.));
#4829=CARTESIAN_POINT('Origin',(0.,-1.73472347597681E-14,10.));
#4830=CARTESIAN_POINT('Origin',(0.,-3.08148791101958E-30,0.));
#5636=UNCERTAINTY_MEASURE_WITH_UNIT(LENGTH_MEASURE(0.01),#5659,
'DISTANCE_ACCURACY_VALUE',
'Maximum model space distance between geometric entities at asserted c
onnectivities');
#5645=UNCERTAINTY_MEASURE_WITH_UNIT(LENGTH_MEASURE(0.01),#5659,
'DISTANCE_ACCURACY_VALUE',
'Maximum model space distance between geometric entities at asserted c
onnectivities');
#5649=(
GEOMETRIC_REPRESENTATION_CONTEXT(3)
GLOBAL_UNCERTAINTY_ASSIGNED_CONTEXT((#5636))
GLOBAL_UNIT_ASSIGNED_CONTEXT((#5659,#5661,#5662))
REPRESENTATION_CONTEXT('','3D')
);
#5658=(
GEOMETRIC_REPRESENTATION_CONTEXT(3)
GLOBAL_UNCERTAINTY_ASSIGNED_CONTEXT((#5645))
GLOBAL_UNIT_ASSIGNED_CONTEXT((#5659,#5661,#5662))
REPRESENTATION_CONTEXT('','3D')
);
#5659=(
LENGTH_UNIT()
NAMED_UNIT(*)
SI_UNIT(.MILLI.,.METRE.)
);
#5661=(
NAMED_UNIT(*)
PLANE_ANGLE_UNIT()
SI_UNIT($,.RADIAN.)
);
#5662=(
NAMED_UNIT(*)
SI_UNIT($,.STERADIAN.)
SOLID_ANGLE_UNIT()
);
#5666=SHAPE_DEFINITION_REPRESENTATION(#5678,#5708);
#5678=PRODUCT_DEFINITION_SHAPE('',$,#5721);
#5708=SHAPE_REPRESENTATION('',(#3240),#5649);
#5717=PRODUCT_DEFINITION_CONTEXT('part definition',#5755,'design');
#5721=PRODUCT_DEFINITION('Camera Arm','Camera Arm',#5733,#5717);
#5733=PRODUCT_DEFINITION_FORMATION('',$,#5760);
#5755=APPLICATION_CONTEXT(
'Core Data for Automotive Mechanical Design Process');
#5756=PRODUCT_CONTEXT('part definition',#5755,'mechanical');
#5760=PRODUCT('Camera Arm','Camera Arm',$,(#5756));
#5772=PRESENTATION_STYLE_ASSIGNMENT((#5777));
#5777=SURFACE_STYLE_USAGE(.BOTH.,#5782);
#5782=SURFACE_SIDE_STYLE('',(#5787));
#5787=SURFACE_STYLE_FILL_AREA(#5792);
#5792=FILL_AREA_STYLE('Opaque(227,224,212)',(#5797));
#5797=FILL_AREA_STYLE_COLOUR('Opaque(227,224,212)',#5802);
#5802=COLOUR_RGB('Opaque(227,224,212)',0.890196078431372,0.87843137254902,
0.831372549019608);
ENDSEC;
END-ISO-10303-21;
